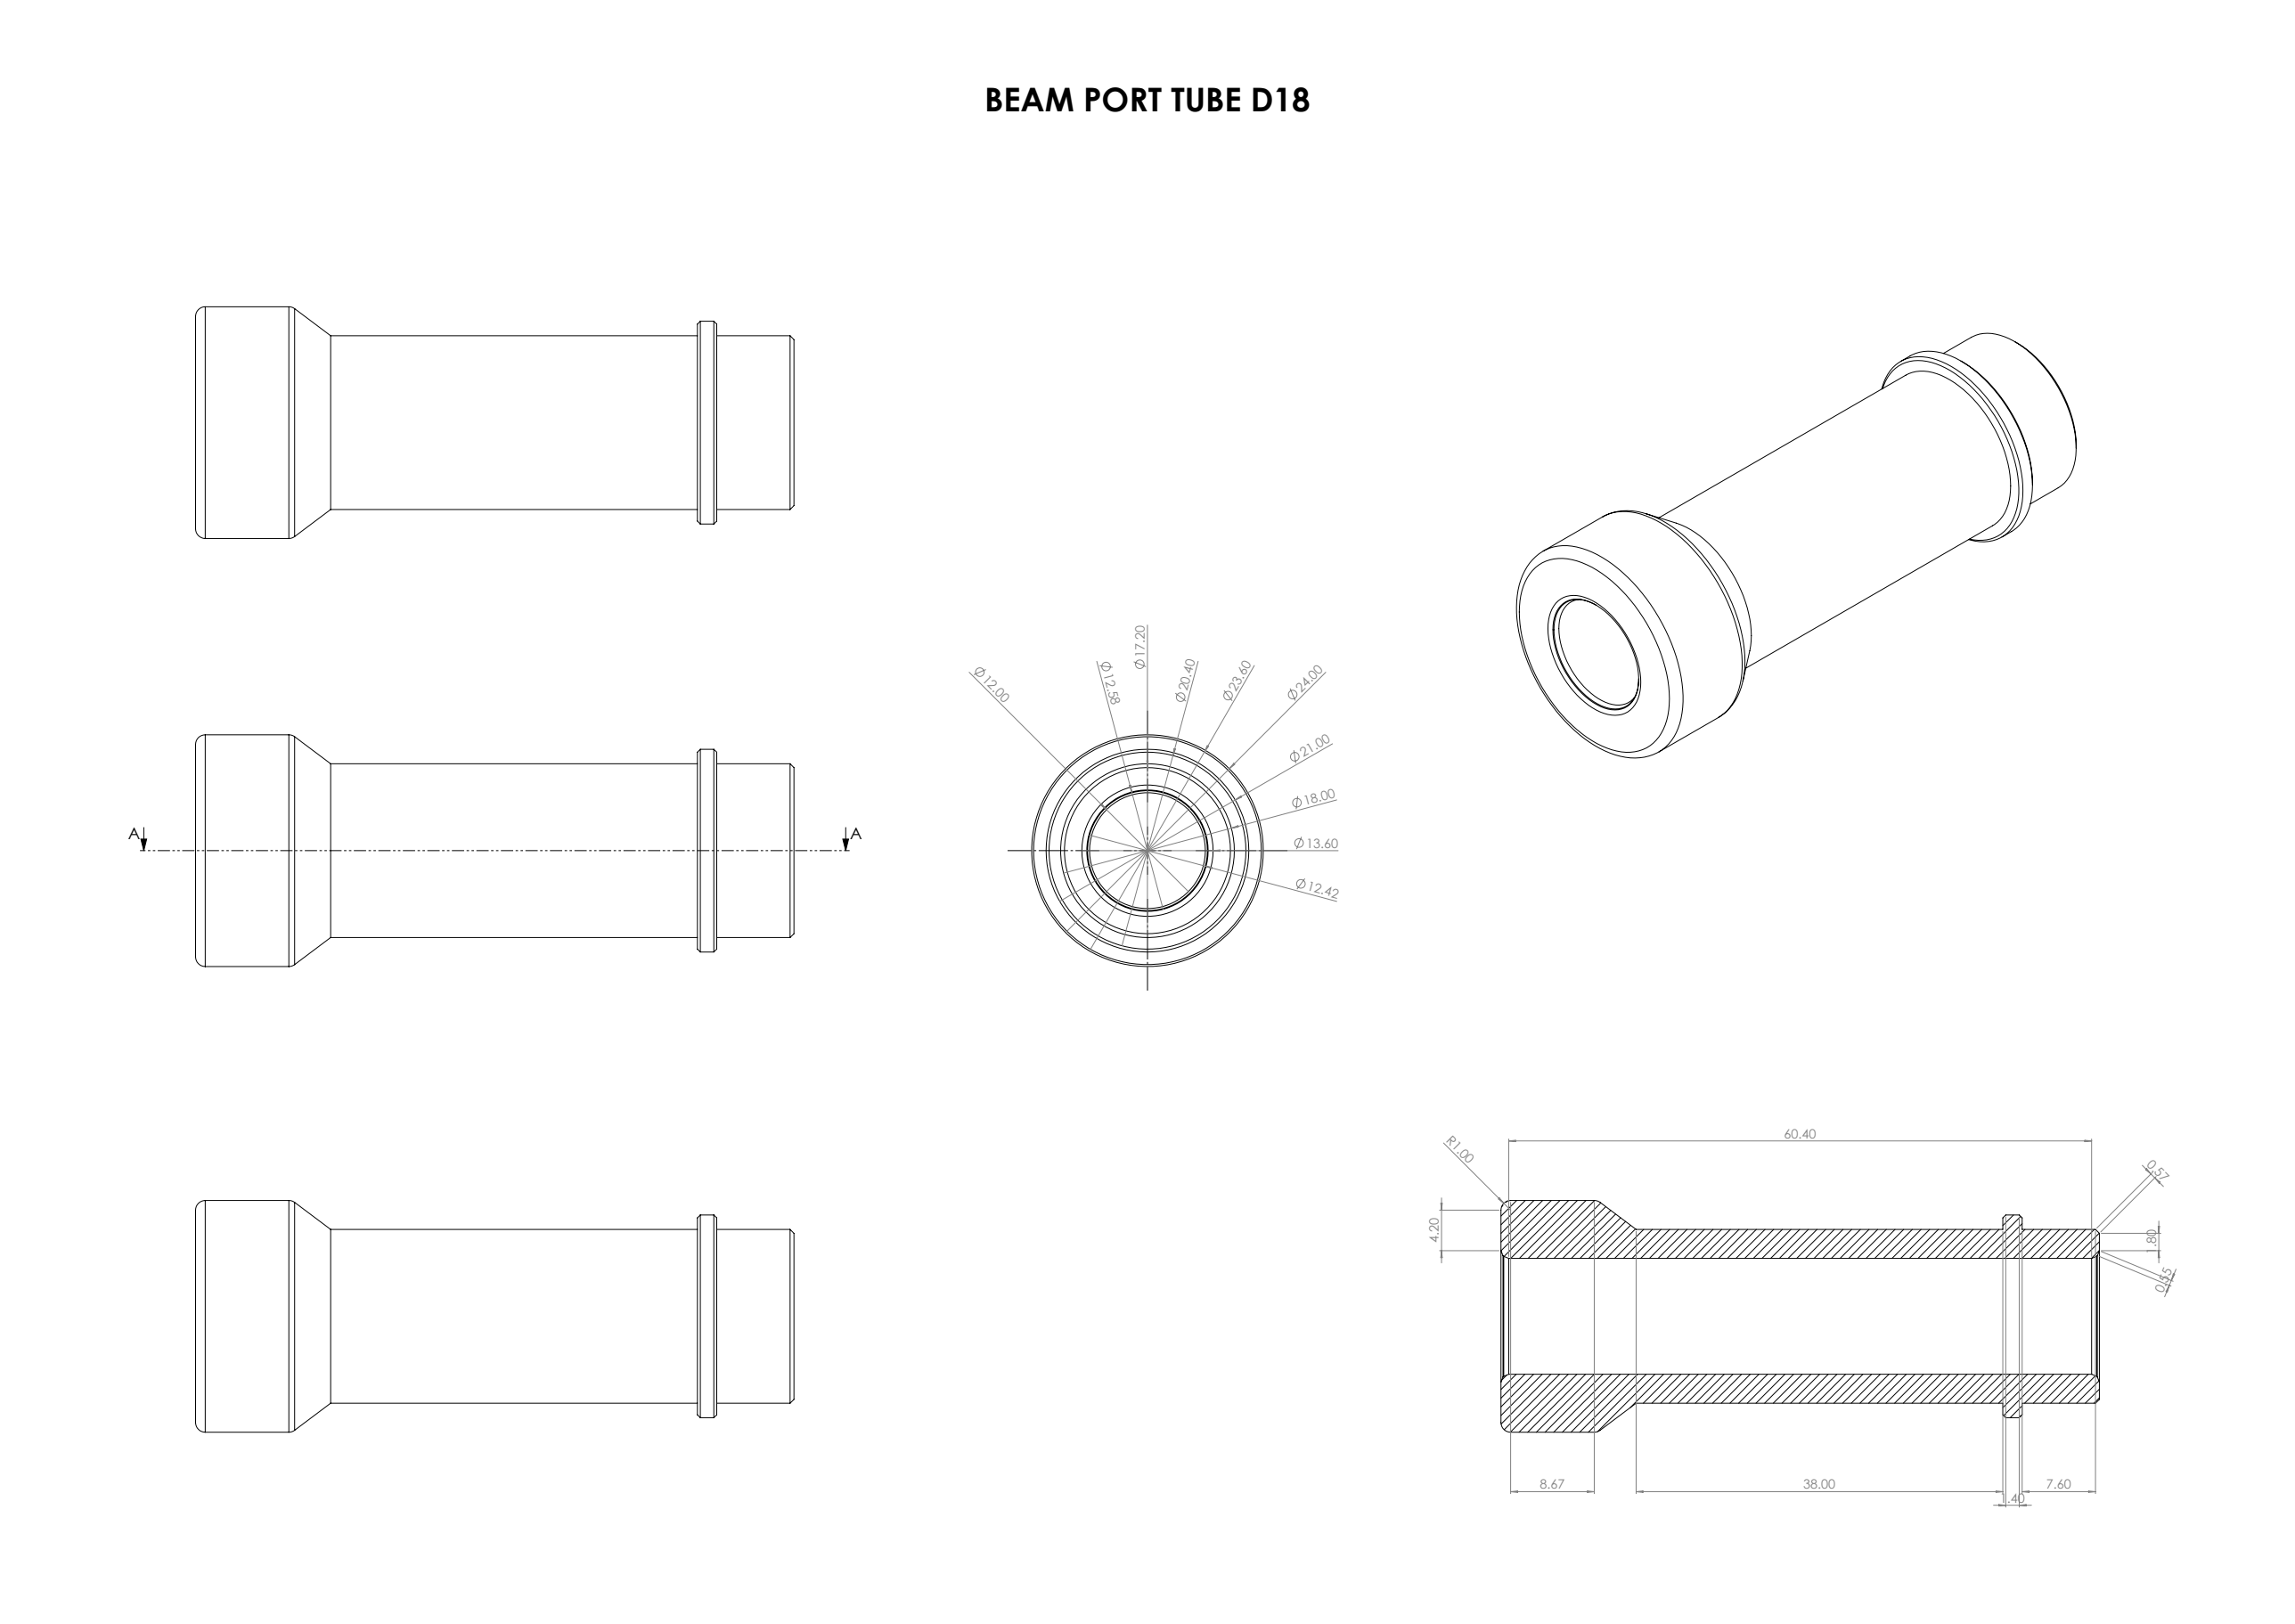
ISO-10303-21;
HEADER;
/* Generated by software containing ST-Developer
 * from STEP Tools, Inc. (www.steptools.com) 
 */

FILE_DESCRIPTION(
/* description */ (''),
/* implementation_level */ '2;1');

FILE_NAME(
/* name */ '04_Beam_Port_Tube_D18.step',
/* time_stamp */ '2026-10-19T23:00:43-07:00',
/* author */ (''),
/* organization */ (''),
/* preprocessor_version */ 'ST-DEVELOPER v20.2',
/* originating_system */ 'Autodesk Translation Framework v15.15.0.0',
/* authorisation */ '');

FILE_SCHEMA (('AUTOMOTIVE_DESIGN { 1 0 10303 214 3 1 1 }'));
ENDSEC;

DATA;
#10=MECHANICAL_DESIGN_GEOMETRIC_PRESENTATION_REPRESENTATION('',(#999),#55002);
#954=TOROIDAL_SURFACE('',#25670,1.1,0.1);
#955=TOROIDAL_SURFACE('',#25675,1.1,0.1);
#959=SHAPE_REPRESENTATION_RELATIONSHIP('SRR','None',#55107,#979);
#979=ADVANCED_BREP_SHAPE_REPRESENTATION('',(#1019),#54985);
#999=STYLED_ITEM('',(#55400),#1019);
#1019=MANIFOLD_SOLID_BREP('Beam Port Tube',#24532);
#1158=FACE_BOUND('',#4320,.T.);
#1159=FACE_BOUND('',#4323,.T.);
#1160=FACE_BOUND('',#4327,.T.);
#1161=FACE_BOUND('',#4334,.T.);
#1414=PLANE('',#25639);
#1415=PLANE('',#25643);
#1416=PLANE('',#25650);
#1417=PLANE('',#25664);
#2116=CYLINDRICAL_SURFACE('',#25636,1.05);
#2117=CYLINDRICAL_SURFACE('',#25655,0.6);
#2118=CYLINDRICAL_SURFACE('',#25669,0.9);
#2119=CYLINDRICAL_SURFACE('',#25673,1.2);
#2120=CYLINDRICAL_SURFACE('',#25680,0.9);
#2831=FACE_OUTER_BOUND('',#4317,.T.);
#2832=FACE_OUTER_BOUND('',#4318,.T.);
#2833=FACE_OUTER_BOUND('',#4319,.T.);
#2834=FACE_OUTER_BOUND('',#4321,.T.);
#2835=FACE_OUTER_BOUND('',#4322,.T.);
#2836=FACE_OUTER_BOUND('',#4324,.T.);
#2837=FACE_OUTER_BOUND('',#4325,.T.);
#2838=FACE_OUTER_BOUND('',#4326,.T.);
#2839=FACE_OUTER_BOUND('',#4328,.T.);
#2840=FACE_OUTER_BOUND('',#4329,.T.);
#2841=FACE_OUTER_BOUND('',#4330,.T.);
#2842=FACE_OUTER_BOUND('',#4331,.T.);
#2843=FACE_OUTER_BOUND('',#4332,.T.);
#2844=FACE_OUTER_BOUND('',#4333,.T.);
#2845=FACE_OUTER_BOUND('',#4335,.T.);
#2846=FACE_OUTER_BOUND('',#4336,.T.);
#2847=FACE_OUTER_BOUND('',#4337,.T.);
#2848=FACE_OUTER_BOUND('',#4338,.T.);
#2849=FACE_OUTER_BOUND('',#4339,.T.);
#2850=FACE_OUTER_BOUND('',#4340,.T.);
#2851=FACE_OUTER_BOUND('',#4341,.T.);
#4317=EDGE_LOOP('',(#17792,#17793,#17794,#17795,#17796));
#4318=EDGE_LOOP('',(#17797,#17798,#17799,#17800,#17801,#17802));
#4319=EDGE_LOOP('',(#17803));
#4320=EDGE_LOOP('',(#17804));
#4321=EDGE_LOOP('',(#17805,#17806,#17807,#17808,#17809));
#4322=EDGE_LOOP('',(#17810));
#4323=EDGE_LOOP('',(#17811));
#4324=EDGE_LOOP('',(#17812,#17813,#17814,#17815));
#4325=EDGE_LOOP('',(#17816,#17817,#17818,#17819));
#4326=EDGE_LOOP('',(#17820));
#4327=EDGE_LOOP('',(#17821));
#4328=EDGE_LOOP('',(#17822,#17823,#17824,#17825,#17826));
#4329=EDGE_LOOP('',(#17827,#17828,#17829,#17830,#17831,#17832));
#4330=EDGE_LOOP('',(#17833,#17834,#17835,#17836,#17837));
#4331=EDGE_LOOP('',(#17838,#17839,#17840,#17841));
#4332=EDGE_LOOP('',(#17842,#17843,#17844,#17845));
#4333=EDGE_LOOP('',(#17846));
#4334=EDGE_LOOP('',(#17847));
#4335=EDGE_LOOP('',(#17848,#17849,#17850,#17851,#17852));
#4336=EDGE_LOOP('',(#17853,#17854,#17855,#17856,#17857));
#4337=EDGE_LOOP('',(#17858,#17859,#17860,#17861));
#4338=EDGE_LOOP('',(#17862,#17863,#17864,#17865));
#4339=EDGE_LOOP('',(#17866,#17867,#17868,#17869));
#4340=EDGE_LOOP('',(#17870,#17871,#17872,#17873));
#4341=EDGE_LOOP('',(#17874,#17875,#17876,#17877));
#5895=LINE('',#35870,#7716);
#5896=LINE('',#35876,#7717);
#5897=LINE('',#35885,#7718);
#5898=LINE('',#35894,#7719);
#5899=LINE('',#35899,#7720);
#5900=LINE('',#35905,#7721);
#5901=LINE('',#35911,#7722);
#5902=LINE('',#35918,#7723);
#5903=LINE('',#35922,#7724);
#5904=LINE('',#35925,#7725);
#5905=LINE('',#35935,#7726);
#5906=LINE('',#35937,#7727);
#5907=LINE('',#35944,#7728);
#5908=LINE('',#35952,#7729);
#5909=LINE('',#35955,#7730);
#7716=VECTOR('',#29439,1.035);
#7717=VECTOR('',#29446,1.05);
#7718=VECTOR('',#29457,1.035);
#7719=VECTOR('',#29468,0.6543933982822);
#7720=VECTOR('',#29475,0.625);
#7721=VECTOR('',#29482,0.610606601717797);
#7722=VECTOR('',#29489,0.6);
#7723=VECTOR('',#29498,0.610606601717798);
#7724=VECTOR('',#29503,0.625);
#7725=VECTOR('',#29506,0.654393398282201);
#7726=VECTOR('',#29519,0.88);
#7727=VECTOR('',#29522,0.9);
#7728=VECTOR('',#29531,1.2);
#7729=VECTOR('',#29542,1.05);
#7730=VECTOR('',#29547,0.9);
#9460=CIRCLE('',#25633,1.02);
#9461=CIRCLE('',#25634,1.05);
#9462=CIRCLE('',#25635,1.05);
#9463=CIRCLE('',#25637,1.05);
#9464=CIRCLE('',#25638,1.05);
#9465=CIRCLE('',#25640,0.9);
#9466=CIRCLE('',#25642,1.02);
#9467=CIRCLE('',#25644,0.9);
#9468=CIRCLE('',#25646,0.628786796564401);
#9469=CIRCLE('',#25647,0.679999999999998);
#9470=CIRCLE('',#25649,0.621213203435595);
#9471=CIRCLE('',#25651,1.1);
#9472=CIRCLE('',#25653,0.6);
#9473=CIRCLE('',#25654,0.6);
#9474=CIRCLE('',#25656,0.6);
#9475=CIRCLE('',#25657,0.6);
#9476=CIRCLE('',#25659,0.621213203435596);
#9477=CIRCLE('',#25661,0.628786796564403);
#9478=CIRCLE('',#25663,0.68);
#9479=CIRCLE('',#25665,0.86);
#9480=CIRCLE('',#25667,0.9);
#9481=CIRCLE('',#25668,0.9);
#9482=CIRCLE('',#25671,0.1);
#9483=CIRCLE('',#25672,1.2);
#9484=CIRCLE('',#25674,1.2);
#9485=CIRCLE('',#25676,0.1);
#9486=CIRCLE('',#25677,1.18);
#9487=CIRCLE('',#25679,0.9);
#10646=VERTEX_POINT('',#35867);
#10647=VERTEX_POINT('',#35869);
#10648=VERTEX_POINT('',#35871);
#10649=VERTEX_POINT('',#35875);
#10650=VERTEX_POINT('',#35877);
#10651=VERTEX_POINT('',#35881);
#10652=VERTEX_POINT('',#35884);
#10653=VERTEX_POINT('',#35888);
#10654=VERTEX_POINT('',#35891);
#10655=VERTEX_POINT('',#35893);
#10656=VERTEX_POINT('',#35897);
#10657=VERTEX_POINT('',#35901);
#10658=VERTEX_POINT('',#35904);
#10659=VERTEX_POINT('',#35906);
#10660=VERTEX_POINT('',#35910);
#10661=VERTEX_POINT('',#35912);
#10662=VERTEX_POINT('',#35916);
#10663=VERTEX_POINT('',#35920);
#10664=VERTEX_POINT('',#35924);
#10665=VERTEX_POINT('',#35928);
#10666=VERTEX_POINT('',#35931);
#10667=VERTEX_POINT('',#35932);
#10668=VERTEX_POINT('',#35939);
#10669=VERTEX_POINT('',#35943);
#10670=VERTEX_POINT('',#35947);
#10671=VERTEX_POINT('',#35951);
#13304=EDGE_CURVE('',#10646,#10646,#9460,.T.);
#13305=EDGE_CURVE('',#10646,#10647,#5895,.T.);
#13306=EDGE_CURVE('',#10647,#10648,#9461,.T.);
#13307=EDGE_CURVE('',#10648,#10647,#9462,.T.);
#13308=EDGE_CURVE('',#10648,#10649,#5896,.T.);
#13309=EDGE_CURVE('',#10650,#10649,#9463,.T.);
#13310=EDGE_CURVE('',#10649,#10650,#9464,.T.);
#13311=EDGE_CURVE('',#10651,#10651,#9465,.T.);
#13312=EDGE_CURVE('',#10650,#10652,#5897,.T.);
#13313=EDGE_CURVE('',#10652,#10652,#9466,.T.);
#13314=EDGE_CURVE('',#10653,#10653,#9467,.T.);
#13315=EDGE_CURVE('',#10654,#10654,#9468,.T.);
#13316=EDGE_CURVE('',#10654,#10655,#5898,.T.);
#13317=EDGE_CURVE('',#10655,#10655,#9469,.T.);
#13318=EDGE_CURVE('',#10656,#10656,#9470,.T.);
#13319=EDGE_CURVE('',#10656,#10654,#5899,.T.);
#13320=EDGE_CURVE('',#10657,#10657,#9471,.T.);
#13321=EDGE_CURVE('',#10656,#10658,#5900,.T.);
#13322=EDGE_CURVE('',#10658,#10659,#9472,.T.);
#13323=EDGE_CURVE('',#10659,#10658,#9473,.T.);
#13324=EDGE_CURVE('',#10659,#10660,#5901,.T.);
#13325=EDGE_CURVE('',#10661,#10660,#9474,.T.);
#13326=EDGE_CURVE('',#10660,#10661,#9475,.T.);
#13327=EDGE_CURVE('',#10662,#10662,#9476,.T.);
#13328=EDGE_CURVE('',#10662,#10661,#5902,.T.);
#13329=EDGE_CURVE('',#10663,#10663,#9477,.T.);
#13330=EDGE_CURVE('',#10663,#10662,#5903,.T.);
#13331=EDGE_CURVE('',#10663,#10664,#5904,.T.);
#13332=EDGE_CURVE('',#10664,#10664,#9478,.T.);
#13333=EDGE_CURVE('',#10665,#10665,#9479,.T.);
#13334=EDGE_CURVE('',#10666,#10667,#9480,.T.);
#13335=EDGE_CURVE('',#10667,#10666,#9481,.T.);
#13336=EDGE_CURVE('',#10666,#10665,#5905,.T.);
#13337=EDGE_CURVE('',#10653,#10667,#5906,.T.);
#13338=EDGE_CURVE('',#10657,#10668,#9482,.T.);
#13339=EDGE_CURVE('',#10668,#10668,#9483,.T.);
#13340=EDGE_CURVE('',#10668,#10669,#5907,.T.);
#13341=EDGE_CURVE('',#10669,#10669,#9484,.T.);
#13342=EDGE_CURVE('',#10669,#10670,#9485,.T.);
#13343=EDGE_CURVE('',#10670,#10670,#9486,.T.);
#13344=EDGE_CURVE('',#10670,#10671,#5908,.T.);
#13345=EDGE_CURVE('',#10671,#10671,#9487,.T.);
#13346=EDGE_CURVE('',#10671,#10651,#5909,.T.);
#17792=ORIENTED_EDGE('',*,*,#13304,.T.);
#17793=ORIENTED_EDGE('',*,*,#13305,.T.);
#17794=ORIENTED_EDGE('',*,*,#13306,.T.);
#17795=ORIENTED_EDGE('',*,*,#13307,.T.);
#17796=ORIENTED_EDGE('',*,*,#13305,.F.);
#17797=ORIENTED_EDGE('',*,*,#13306,.F.);
#17798=ORIENTED_EDGE('',*,*,#13307,.F.);
#17799=ORIENTED_EDGE('',*,*,#13308,.T.);
#17800=ORIENTED_EDGE('',*,*,#13309,.F.);
#17801=ORIENTED_EDGE('',*,*,#13310,.F.);
#17802=ORIENTED_EDGE('',*,*,#13308,.F.);
#17803=ORIENTED_EDGE('',*,*,#13304,.F.);
#17804=ORIENTED_EDGE('',*,*,#13311,.F.);
#17805=ORIENTED_EDGE('',*,*,#13309,.T.);
#17806=ORIENTED_EDGE('',*,*,#13310,.T.);
#17807=ORIENTED_EDGE('',*,*,#13312,.T.);
#17808=ORIENTED_EDGE('',*,*,#13313,.T.);
#17809=ORIENTED_EDGE('',*,*,#13312,.F.);
#17810=ORIENTED_EDGE('',*,*,#13313,.F.);
#17811=ORIENTED_EDGE('',*,*,#13314,.T.);
#17812=ORIENTED_EDGE('',*,*,#13315,.T.);
#17813=ORIENTED_EDGE('',*,*,#13316,.T.);
#17814=ORIENTED_EDGE('',*,*,#13317,.T.);
#17815=ORIENTED_EDGE('',*,*,#13316,.F.);
#17816=ORIENTED_EDGE('',*,*,#13318,.F.);
#17817=ORIENTED_EDGE('',*,*,#13319,.T.);
#17818=ORIENTED_EDGE('',*,*,#13315,.F.);
#17819=ORIENTED_EDGE('',*,*,#13319,.F.);
#17820=ORIENTED_EDGE('',*,*,#13320,.F.);
#17821=ORIENTED_EDGE('',*,*,#13317,.F.);
#17822=ORIENTED_EDGE('',*,*,#13318,.T.);
#17823=ORIENTED_EDGE('',*,*,#13321,.T.);
#17824=ORIENTED_EDGE('',*,*,#13322,.T.);
#17825=ORIENTED_EDGE('',*,*,#13323,.T.);
#17826=ORIENTED_EDGE('',*,*,#13321,.F.);
#17827=ORIENTED_EDGE('',*,*,#13322,.F.);
#17828=ORIENTED_EDGE('',*,*,#13323,.F.);
#17829=ORIENTED_EDGE('',*,*,#13324,.T.);
#17830=ORIENTED_EDGE('',*,*,#13325,.F.);
#17831=ORIENTED_EDGE('',*,*,#13326,.F.);
#17832=ORIENTED_EDGE('',*,*,#13324,.F.);
#17833=ORIENTED_EDGE('',*,*,#13327,.T.);
#17834=ORIENTED_EDGE('',*,*,#13328,.T.);
#17835=ORIENTED_EDGE('',*,*,#13325,.T.);
#17836=ORIENTED_EDGE('',*,*,#13326,.T.);
#17837=ORIENTED_EDGE('',*,*,#13328,.F.);
#17838=ORIENTED_EDGE('',*,*,#13329,.F.);
#17839=ORIENTED_EDGE('',*,*,#13330,.T.);
#17840=ORIENTED_EDGE('',*,*,#13327,.F.);
#17841=ORIENTED_EDGE('',*,*,#13330,.F.);
#17842=ORIENTED_EDGE('',*,*,#13329,.T.);
#17843=ORIENTED_EDGE('',*,*,#13331,.T.);
#17844=ORIENTED_EDGE('',*,*,#13332,.T.);
#17845=ORIENTED_EDGE('',*,*,#13331,.F.);
#17846=ORIENTED_EDGE('',*,*,#13333,.F.);
#17847=ORIENTED_EDGE('',*,*,#13332,.F.);
#17848=ORIENTED_EDGE('',*,*,#13334,.T.);
#17849=ORIENTED_EDGE('',*,*,#13335,.T.);
#17850=ORIENTED_EDGE('',*,*,#13336,.T.);
#17851=ORIENTED_EDGE('',*,*,#13333,.T.);
#17852=ORIENTED_EDGE('',*,*,#13336,.F.);
#17853=ORIENTED_EDGE('',*,*,#13314,.F.);
#17854=ORIENTED_EDGE('',*,*,#13337,.T.);
#17855=ORIENTED_EDGE('',*,*,#13334,.F.);
#17856=ORIENTED_EDGE('',*,*,#13335,.F.);
#17857=ORIENTED_EDGE('',*,*,#13337,.F.);
#17858=ORIENTED_EDGE('',*,*,#13320,.T.);
#17859=ORIENTED_EDGE('',*,*,#13338,.T.);
#17860=ORIENTED_EDGE('',*,*,#13339,.T.);
#17861=ORIENTED_EDGE('',*,*,#13338,.F.);
#17862=ORIENTED_EDGE('',*,*,#13339,.F.);
#17863=ORIENTED_EDGE('',*,*,#13340,.T.);
#17864=ORIENTED_EDGE('',*,*,#13341,.F.);
#17865=ORIENTED_EDGE('',*,*,#13340,.F.);
#17866=ORIENTED_EDGE('',*,*,#13341,.T.);
#17867=ORIENTED_EDGE('',*,*,#13342,.T.);
#17868=ORIENTED_EDGE('',*,*,#13343,.T.);
#17869=ORIENTED_EDGE('',*,*,#13342,.F.);
#17870=ORIENTED_EDGE('',*,*,#13343,.F.);
#17871=ORIENTED_EDGE('',*,*,#13344,.T.);
#17872=ORIENTED_EDGE('',*,*,#13345,.T.);
#17873=ORIENTED_EDGE('',*,*,#13344,.F.);
#17874=ORIENTED_EDGE('',*,*,#13345,.F.);
#17875=ORIENTED_EDGE('',*,*,#13346,.T.);
#17876=ORIENTED_EDGE('',*,*,#13311,.T.);
#17877=ORIENTED_EDGE('',*,*,#13346,.F.);
#23073=CONICAL_SURFACE('',#25632,1.035,0.785398163397459);
#23074=CONICAL_SURFACE('',#25641,1.035,0.785398163397459);
#23075=CONICAL_SURFACE('',#25645,0.6543933982822,1.17809724509617);
#23076=CONICAL_SURFACE('',#25648,0.625,0.785398163397442);
#23077=CONICAL_SURFACE('',#25652,0.610606601717797,0.39269908169869);
#23078=CONICAL_SURFACE('',#25658,0.610606601717798,0.392699081698726);
#23079=CONICAL_SURFACE('',#25660,0.625,0.785398163397442);
#23080=CONICAL_SURFACE('',#25662,0.654393398282201,1.17809724509617);
#23081=CONICAL_SURFACE('',#25666,0.88,0.785398163397459);
#23082=CONICAL_SURFACE('',#25678,1.05,0.643501108793286);
#23584=ADVANCED_FACE('',(#2831),#23073,.T.);
#23585=ADVANCED_FACE('',(#2832),#2116,.T.);
#23586=ADVANCED_FACE('',(#2833,#1158),#1414,.T.);
#23587=ADVANCED_FACE('',(#2834),#23074,.T.);
#23588=ADVANCED_FACE('',(#2835,#1159),#1415,.T.);
#23589=ADVANCED_FACE('',(#2836),#23075,.F.);
#23590=ADVANCED_FACE('',(#2837),#23076,.F.);
#23591=ADVANCED_FACE('',(#2838,#1160),#1416,.T.);
#23592=ADVANCED_FACE('',(#2839),#23077,.F.);
#23593=ADVANCED_FACE('',(#2840),#2117,.F.);
#23594=ADVANCED_FACE('',(#2841),#23078,.F.);
#23595=ADVANCED_FACE('',(#2842),#23079,.F.);
#23596=ADVANCED_FACE('',(#2843),#23080,.F.);
#23597=ADVANCED_FACE('',(#2844,#1161),#1417,.T.);
#23598=ADVANCED_FACE('',(#2845),#23081,.T.);
#23599=ADVANCED_FACE('',(#2846),#2118,.T.);
#23600=ADVANCED_FACE('',(#2847),#954,.T.);
#23601=ADVANCED_FACE('',(#2848),#2119,.T.);
#23602=ADVANCED_FACE('',(#2849),#955,.T.);
#23603=ADVANCED_FACE('',(#2850),#23082,.T.);
#23604=ADVANCED_FACE('',(#2851),#2120,.T.);
#24532=CLOSED_SHELL('',(#23584,#23585,#23586,#23587,#23588,#23589,#23590,
#23591,#23592,#23593,#23594,#23595,#23596,#23597,#23598,#23599,#23600,#23601,
#23602,#23603,#23604));
#25631=AXIS2_PLACEMENT_3D('',#35865,#29433,#29434);
#25632=AXIS2_PLACEMENT_3D('',#35866,#29435,#29436);
#25633=AXIS2_PLACEMENT_3D('',#35868,#29437,#29438);
#25634=AXIS2_PLACEMENT_3D('',#35872,#29440,#29441);
#25635=AXIS2_PLACEMENT_3D('',#35873,#29442,#29443);
#25636=AXIS2_PLACEMENT_3D('',#35874,#29444,#29445);
#25637=AXIS2_PLACEMENT_3D('',#35878,#29447,#29448);
#25638=AXIS2_PLACEMENT_3D('',#35879,#29449,#29450);
#25639=AXIS2_PLACEMENT_3D('',#35880,#29451,#29452);
#25640=AXIS2_PLACEMENT_3D('',#35882,#29453,#29454);
#25641=AXIS2_PLACEMENT_3D('',#35883,#29455,#29456);
#25642=AXIS2_PLACEMENT_3D('',#35886,#29458,#29459);
#25643=AXIS2_PLACEMENT_3D('',#35887,#29460,#29461);
#25644=AXIS2_PLACEMENT_3D('',#35889,#29462,#29463);
#25645=AXIS2_PLACEMENT_3D('',#35890,#29464,#29465);
#25646=AXIS2_PLACEMENT_3D('',#35892,#29466,#29467);
#25647=AXIS2_PLACEMENT_3D('',#35895,#29469,#29470);
#25648=AXIS2_PLACEMENT_3D('',#35896,#29471,#29472);
#25649=AXIS2_PLACEMENT_3D('',#35898,#29473,#29474);
#25650=AXIS2_PLACEMENT_3D('',#35900,#29476,#29477);
#25651=AXIS2_PLACEMENT_3D('',#35902,#29478,#29479);
#25652=AXIS2_PLACEMENT_3D('',#35903,#29480,#29481);
#25653=AXIS2_PLACEMENT_3D('',#35907,#29483,#29484);
#25654=AXIS2_PLACEMENT_3D('',#35908,#29485,#29486);
#25655=AXIS2_PLACEMENT_3D('',#35909,#29487,#29488);
#25656=AXIS2_PLACEMENT_3D('',#35913,#29490,#29491);
#25657=AXIS2_PLACEMENT_3D('',#35914,#29492,#29493);
#25658=AXIS2_PLACEMENT_3D('',#35915,#29494,#29495);
#25659=AXIS2_PLACEMENT_3D('',#35917,#29496,#29497);
#25660=AXIS2_PLACEMENT_3D('',#35919,#29499,#29500);
#25661=AXIS2_PLACEMENT_3D('',#35921,#29501,#29502);
#25662=AXIS2_PLACEMENT_3D('',#35923,#29504,#29505);
#25663=AXIS2_PLACEMENT_3D('',#35926,#29507,#29508);
#25664=AXIS2_PLACEMENT_3D('',#35927,#29509,#29510);
#25665=AXIS2_PLACEMENT_3D('',#35929,#29511,#29512);
#25666=AXIS2_PLACEMENT_3D('',#35930,#29513,#29514);
#25667=AXIS2_PLACEMENT_3D('',#35933,#29515,#29516);
#25668=AXIS2_PLACEMENT_3D('',#35934,#29517,#29518);
#25669=AXIS2_PLACEMENT_3D('',#35936,#29520,#29521);
#25670=AXIS2_PLACEMENT_3D('',#35938,#29523,#29524);
#25671=AXIS2_PLACEMENT_3D('',#35940,#29525,#29526);
#25672=AXIS2_PLACEMENT_3D('',#35941,#29527,#29528);
#25673=AXIS2_PLACEMENT_3D('',#35942,#29529,#29530);
#25674=AXIS2_PLACEMENT_3D('',#35945,#29532,#29533);
#25675=AXIS2_PLACEMENT_3D('',#35946,#29534,#29535);
#25676=AXIS2_PLACEMENT_3D('',#35948,#29536,#29537);
#25677=AXIS2_PLACEMENT_3D('',#35949,#29538,#29539);
#25678=AXIS2_PLACEMENT_3D('',#35950,#29540,#29541);
#25679=AXIS2_PLACEMENT_3D('',#35953,#29543,#29544);
#25680=AXIS2_PLACEMENT_3D('',#35954,#29545,#29546);
#29433=DIRECTION('axis',(0.,0.,1.));
#29434=DIRECTION('refdir',(1.,0.,0.));
#29435=DIRECTION('center_axis',(0.,0.,-1.));
#29436=DIRECTION('ref_axis',(-1.,0.,0.));
#29437=DIRECTION('center_axis',(0.,0.,-1.));
#29438=DIRECTION('ref_axis',(-1.,0.,0.));
#29439=DIRECTION('',(0.707106781186555,8.65956056235503E-17,-0.70710678118654));
#29440=DIRECTION('center_axis',(0.,0.,1.));
#29441=DIRECTION('ref_axis',(-1.,0.,0.));
#29442=DIRECTION('center_axis',(0.,0.,1.));
#29443=DIRECTION('ref_axis',(-1.,0.,0.));
#29444=DIRECTION('center_axis',(0.,0.,1.));
#29445=DIRECTION('ref_axis',(1.,0.,0.));
#29446=DIRECTION('',(0.,0.,-1.));
#29447=DIRECTION('center_axis',(0.,0.,-1.));
#29448=DIRECTION('ref_axis',(-1.,0.,0.));
#29449=DIRECTION('center_axis',(0.,0.,-1.));
#29450=DIRECTION('ref_axis',(-1.,0.,0.));
#29451=DIRECTION('center_axis',(0.,0.,1.));
#29452=DIRECTION('ref_axis',(1.,0.,0.));
#29453=DIRECTION('center_axis',(0.,0.,1.));
#29454=DIRECTION('ref_axis',(1.,0.,0.));
#29455=DIRECTION('center_axis',(0.,0.,1.));
#29456=DIRECTION('ref_axis',(-1.,0.,0.));
#29457=DIRECTION('',(-0.707106781186555,-8.65956056235503E-17,-0.70710678118654));
#29458=DIRECTION('center_axis',(0.,0.,1.));
#29459=DIRECTION('ref_axis',(-1.,0.,0.));
#29460=DIRECTION('center_axis',(0.,0.,-1.));
#29461=DIRECTION('ref_axis',(-1.,0.,0.));
#29462=DIRECTION('center_axis',(0.,0.,1.));
#29463=DIRECTION('ref_axis',(1.,0.,0.));
#29464=DIRECTION('center_axis',(0.,1.81500578188617E-15,1.));
#29465=DIRECTION('ref_axis',(-1.,2.94181504497177E-17,0.));
#29466=DIRECTION('center_axis',(0.,0.,-1.));
#29467=DIRECTION('ref_axis',(-1.,6.12323399573677E-17,0.));
#29468=DIRECTION('',(0.923879532511288,5.54251204061075E-16,0.382683432365087));
#29469=DIRECTION('center_axis',(0.,0.,1.));
#29470=DIRECTION('ref_axis',(-1.,0.,0.));
#29471=DIRECTION('center_axis',(0.,0.,1.));
#29472=DIRECTION('ref_axis',(-1.,0.,0.));
#29473=DIRECTION('center_axis',(0.,0.,1.));
#29474=DIRECTION('ref_axis',(-1.,6.12323399573677E-17,0.));
#29475=DIRECTION('',(0.707106781186543,-8.65956056235487E-17,0.707106781186552));
#29476=DIRECTION('center_axis',(0.,0.,1.));
#29477=DIRECTION('ref_axis',(1.,0.,0.));
#29478=DIRECTION('center_axis',(0.,0.,-1.));
#29479=DIRECTION('ref_axis',(-1.,1.22464679914735E-16,0.));
#29480=DIRECTION('center_axis',(0.,-7.42744751489879E-16,1.));
#29481=DIRECTION('ref_axis',(-1.,3.11479911548302E-17,0.));
#29482=DIRECTION('',(-0.382683432365058,6.51261289894839E-16,-0.9238795325113));
#29483=DIRECTION('center_axis',(0.,0.,-1.));
#29484=DIRECTION('ref_axis',(-1.,0.,0.));
#29485=DIRECTION('center_axis',(0.,0.,-1.));
#29486=DIRECTION('ref_axis',(-1.,0.,0.));
#29487=DIRECTION('center_axis',(0.,0.,1.));
#29488=DIRECTION('ref_axis',(1.,0.,0.));
#29489=DIRECTION('',(0.,0.,-1.));
#29490=DIRECTION('center_axis',(0.,0.,1.));
#29491=DIRECTION('ref_axis',(-1.,0.,0.));
#29492=DIRECTION('center_axis',(0.,0.,1.));
#29493=DIRECTION('ref_axis',(-1.,0.,0.));
#29494=DIRECTION('center_axis',(0.,-7.42744751489906E-16,-1.));
#29495=DIRECTION('ref_axis',(-1.,3.11479911548302E-17,0.));
#29496=DIRECTION('center_axis',(0.,0.,-1.));
#29497=DIRECTION('ref_axis',(-1.,6.12323399573677E-17,0.));
#29498=DIRECTION('',(-0.382683432365092,7.44991698001377E-16,0.923879532511286));
#29499=DIRECTION('center_axis',(0.,0.,-1.));
#29500=DIRECTION('ref_axis',(-1.,0.,0.));
#29501=DIRECTION('center_axis',(0.,0.,1.));
#29502=DIRECTION('ref_axis',(-1.,6.12323399573677E-17,0.));
#29503=DIRECTION('',(-0.707106781186543,8.65956056235487E-17,0.707106781186552));
#29504=DIRECTION('center_axis',(0.,1.81500578188617E-15,-1.));
#29505=DIRECTION('ref_axis',(-1.,2.94181504497177E-17,0.));
#29506=DIRECTION('',(0.923879532511285,7.80536426518631E-16,-0.382683432365095));
#29507=DIRECTION('center_axis',(0.,0.,-1.));
#29508=DIRECTION('ref_axis',(-1.,0.,0.));
#29509=DIRECTION('center_axis',(0.,0.,-1.));
#29510=DIRECTION('ref_axis',(-1.,0.,0.));
#29511=DIRECTION('center_axis',(0.,0.,1.));
#29512=DIRECTION('ref_axis',(-1.,0.,0.));
#29513=DIRECTION('center_axis',(0.,0.,1.));
#29514=DIRECTION('ref_axis',(-1.,0.,0.));
#29515=DIRECTION('center_axis',(0.,0.,-1.));
#29516=DIRECTION('ref_axis',(-1.,0.,0.));
#29517=DIRECTION('center_axis',(0.,0.,-1.));
#29518=DIRECTION('ref_axis',(-1.,0.,0.));
#29519=DIRECTION('',(-0.707106781186555,-8.65956056235503E-17,-0.70710678118654));
#29520=DIRECTION('center_axis',(0.,0.,1.));
#29521=DIRECTION('ref_axis',(1.,0.,0.));
#29522=DIRECTION('',(0.,0.,-1.));
#29523=DIRECTION('center_axis',(0.,0.,1.));
#29524=DIRECTION('ref_axis',(1.,0.,0.));
#29525=DIRECTION('center_axis',(1.22464679914735E-16,-1.,0.));
#29526=DIRECTION('ref_axis',(-1.,-1.22464679914735E-16,0.));
#29527=DIRECTION('center_axis',(0.,0.,1.));
#29528=DIRECTION('ref_axis',(-1.,1.22464679914735E-16,0.));
#29529=DIRECTION('center_axis',(0.,0.,1.));
#29530=DIRECTION('ref_axis',(1.,0.,0.));
#29531=DIRECTION('',(0.,0.,-1.));
#29532=DIRECTION('center_axis',(0.,0.,-1.));
#29533=DIRECTION('ref_axis',(-1.,1.22464679914735E-16,0.));
#29534=DIRECTION('center_axis',(0.,0.,1.));
#29535=DIRECTION('ref_axis',(1.,0.,0.));
#29536=DIRECTION('center_axis',(1.22464679914735E-16,-1.,0.));
#29537=DIRECTION('ref_axis',(-1.,-1.22464679914735E-16,0.));
#29538=DIRECTION('center_axis',(0.,0.,1.));
#29539=DIRECTION('ref_axis',(-1.,0.,0.));
#29540=DIRECTION('center_axis',(0.,0.,1.));
#29541=DIRECTION('ref_axis',(1.,0.,0.));
#29542=DIRECTION('',(0.600000000000001,7.34788079488414E-17,-0.799999999999999));
#29543=DIRECTION('center_axis',(0.,0.,1.));
#29544=DIRECTION('ref_axis',(1.,0.,0.));
#29545=DIRECTION('center_axis',(0.,0.,1.));
#29546=DIRECTION('ref_axis',(1.,0.,0.));
#29547=DIRECTION('',(0.,0.,-1.));
#35865=CARTESIAN_POINT('',(0.,0.,0.));
#35866=CARTESIAN_POINT('Origin',(0.,0.,12.785));
#35867=CARTESIAN_POINT('',(1.02,-1.2491397351303E-16,12.8));
#35868=CARTESIAN_POINT('Origin',(0.,0.,12.8));
#35869=CARTESIAN_POINT('',(1.05,1.28587913910472E-16,12.77));
#35870=CARTESIAN_POINT('',(1.035,1.26750943711751E-16,12.785));
#35871=CARTESIAN_POINT('',(-1.05,-1.28587913910472E-16,12.77));
#35872=CARTESIAN_POINT('Origin',(0.,0.,12.77));
#35873=CARTESIAN_POINT('Origin',(0.,0.,12.77));
#35874=CARTESIAN_POINT('Origin',(0.,0.,12.7));
#35875=CARTESIAN_POINT('',(-1.05,-1.28587913910472E-16,12.63));
#35876=CARTESIAN_POINT('',(-1.05,-1.28587913910472E-16,12.7));
#35877=CARTESIAN_POINT('',(1.05,-1.28587913910472E-16,12.63));
#35878=CARTESIAN_POINT('Origin',(0.,0.,12.63));
#35879=CARTESIAN_POINT('Origin',(0.,0.,12.63));
#35880=CARTESIAN_POINT('Origin',(0.9,0.,12.8));
#35881=CARTESIAN_POINT('',(-0.9,-1.10218211923262E-16,12.8));
#35882=CARTESIAN_POINT('Origin',(0.,0.,12.8));
#35883=CARTESIAN_POINT('Origin',(0.,0.,12.615));
#35884=CARTESIAN_POINT('',(1.02,1.2491397351303E-16,12.6));
#35885=CARTESIAN_POINT('',(1.035,1.26750943711751E-16,12.615));
#35886=CARTESIAN_POINT('Origin',(0.,0.,12.6));
#35887=CARTESIAN_POINT('Origin',(1.05,0.,12.6));
#35888=CARTESIAN_POINT('',(-0.9,-1.10218211923262E-16,12.6));
#35889=CARTESIAN_POINT('Origin',(0.,0.,12.6));
#35890=CARTESIAN_POINT('Origin',(0.,-1.92510434439678E-17,17.9893933982822));
#35891=CARTESIAN_POINT('',(0.628786796564401,-1.54008347551742E-16,17.9787867965644));
#35892=CARTESIAN_POINT('Origin',(0.,-3.85020868879356E-17,17.9787867965644));
#35893=CARTESIAN_POINT('',(0.679999999999998,8.32759823420198E-17,18.));
#35894=CARTESIAN_POINT('',(0.6543933982822,-1.18642164946881E-16,17.9893933982822));
#35895=CARTESIAN_POINT('Origin',(0.,0.,18.));
#35896=CARTESIAN_POINT('Origin',(0.,0.,17.975));
#35897=CARTESIAN_POINT('',(0.621213203435595,0.,17.9712132034356));
#35898=CARTESIAN_POINT('Origin',(0.,-3.80383380587737E-17,17.9712132034356));
#35899=CARTESIAN_POINT('',(0.625,-7.65404249467096E-17,17.975));
#35900=CARTESIAN_POINT('Origin',(0.6,0.,18.));
#35901=CARTESIAN_POINT('',(-1.1,-1.34711147906209E-16,18.));
#35902=CARTESIAN_POINT('Origin',(0.,0.,18.));
#35903=CARTESIAN_POINT('Origin',(0.,-1.90191690293869E-17,17.9456066017178));
#35904=CARTESIAN_POINT('',(0.6,-7.34788079488412E-17,17.92));
#35905=CARTESIAN_POINT('',(0.610606601717797,3.67394039744206E-17,17.9456066017178));
#35906=CARTESIAN_POINT('',(-0.6,-7.34788079488412E-17,17.92));
#35907=CARTESIAN_POINT('Origin',(0.,0.,17.92));
#35908=CARTESIAN_POINT('Origin',(0.,0.,17.92));
#35909=CARTESIAN_POINT('Origin',(0.,0.,14.9));
#35910=CARTESIAN_POINT('',(-0.6,-7.34788079488412E-17,11.88));
#35911=CARTESIAN_POINT('',(-0.6,-7.34788079488412E-17,14.9));
#35912=CARTESIAN_POINT('',(0.6,7.34788079488412E-17,11.88));
#35913=CARTESIAN_POINT('Origin',(0.,0.,11.88));
#35914=CARTESIAN_POINT('Origin',(0.,0.,11.88));
#35915=CARTESIAN_POINT('Origin',(0.,-1.90191690293869E-17,11.8543933982822));
#35916=CARTESIAN_POINT('',(0.621213203435596,-1.52153352235095E-16,11.8287867965644));
#35917=CARTESIAN_POINT('Origin',(0.,-3.80383380587738E-17,11.8287867965644));
#35918=CARTESIAN_POINT('',(0.610606601717798,-1.12816080091968E-16,11.8543933982822));
#35919=CARTESIAN_POINT('Origin',(0.,0.,11.825));
#35920=CARTESIAN_POINT('',(0.628786796564403,0.,11.8212132034356));
#35921=CARTESIAN_POINT('Origin',(0.,-3.85020868879357E-17,11.8212132034356));
#35922=CARTESIAN_POINT('',(0.625,-7.65404249467096E-17,11.825));
#35923=CARTESIAN_POINT('Origin',(0.,-1.92510434439679E-17,11.8106066017178));
#35924=CARTESIAN_POINT('',(0.68,-8.327598234202E-17,11.8));
#35925=CARTESIAN_POINT('',(0.654393398282201,4.163799117101E-17,11.8106066017178));
#35926=CARTESIAN_POINT('Origin',(0.,0.,11.8));
#35927=CARTESIAN_POINT('Origin',(0.9,0.,11.8));
#35928=CARTESIAN_POINT('',(0.86,1.05319624726672E-16,11.8));
#35929=CARTESIAN_POINT('Origin',(0.,0.,11.8));
#35930=CARTESIAN_POINT('Origin',(0.,0.,11.82));
#35931=CARTESIAN_POINT('',(0.9,-1.10218211923262E-16,11.84));
#35932=CARTESIAN_POINT('',(-0.9,-1.10218211923262E-16,11.84));
#35933=CARTESIAN_POINT('Origin',(0.,0.,11.84));
#35934=CARTESIAN_POINT('Origin',(0.,0.,11.84));
#35935=CARTESIAN_POINT('',(0.88,1.07768918324967E-16,11.82));
#35936=CARTESIAN_POINT('Origin',(0.,0.,12.2));
#35937=CARTESIAN_POINT('',(-0.9,-1.10218211923262E-16,12.2));
#35938=CARTESIAN_POINT('Origin',(0.,0.,17.9));
#35939=CARTESIAN_POINT('',(-1.2,-1.46957615897682E-16,17.9));
#35940=CARTESIAN_POINT('Origin',(-1.1,-1.34711147906209E-16,17.9));
#35941=CARTESIAN_POINT('Origin',(0.,0.,17.9));
#35942=CARTESIAN_POINT('Origin',(0.,0.,17.5));
#35943=CARTESIAN_POINT('',(-1.2,-1.46957615897682E-16,17.0333333333333));
#35944=CARTESIAN_POINT('',(-1.2,-1.46957615897682E-16,17.5));
#35945=CARTESIAN_POINT('Origin',(0.,0.,17.0333333333333));
#35946=CARTESIAN_POINT('Origin',(0.,0.,17.0333333333333));
#35947=CARTESIAN_POINT('',(-1.18,-1.44508322299388E-16,16.9733333333333));
#35948=CARTESIAN_POINT('Origin',(-1.1,-1.34711147906209E-16,17.0333333333333));
#35949=CARTESIAN_POINT('Origin',(0.,-1.44508322299388E-16,16.9733333333333));
#35950=CARTESIAN_POINT('Origin',(0.,0.,16.8));
#35951=CARTESIAN_POINT('',(-0.9,-1.10218211923262E-16,16.6));
#35952=CARTESIAN_POINT('',(-1.05,-1.28587913910472E-16,16.8));
#35953=CARTESIAN_POINT('Origin',(0.,0.,16.6));
#35954=CARTESIAN_POINT('Origin',(0.,0.,14.7));
#35955=CARTESIAN_POINT('',(-0.9,-1.10218211923262E-16,14.7));
#54963=UNCERTAINTY_MEASURE_WITH_UNIT(LENGTH_MEASURE(0.001),#55003,
'DISTANCE_ACCURACY_VALUE',
'Maximum model space distance between geometric entities at asserted c
onnectivities');
#54980=UNCERTAINTY_MEASURE_WITH_UNIT(LENGTH_MEASURE(0.001),#55003,
'DISTANCE_ACCURACY_VALUE',
'Maximum model space distance between geometric entities at asserted c
onnectivities');
#54985=(
GEOMETRIC_REPRESENTATION_CONTEXT(3)
GLOBAL_UNCERTAINTY_ASSIGNED_CONTEXT((#54963))
GLOBAL_UNIT_ASSIGNED_CONTEXT((#55003,#55005,#55006))
REPRESENTATION_CONTEXT('','3D')
);
#55002=(
GEOMETRIC_REPRESENTATION_CONTEXT(3)
GLOBAL_UNCERTAINTY_ASSIGNED_CONTEXT((#54980))
GLOBAL_UNIT_ASSIGNED_CONTEXT((#55003,#55005,#55006))
REPRESENTATION_CONTEXT('','3D')
);
#55003=(
LENGTH_UNIT()
NAMED_UNIT(*)
SI_UNIT(.CENTI.,.METRE.)
);
#55005=(
NAMED_UNIT(*)
PLANE_ANGLE_UNIT()
SI_UNIT($,.RADIAN.)
);
#55006=(
NAMED_UNIT(*)
SI_UNIT($,.STERADIAN.)
SOLID_ANGLE_UNIT()
);
#55011=SHAPE_DEFINITION_REPRESENTATION(#55032,#55107);
#55032=PRODUCT_DEFINITION_SHAPE('',$,#55129);
#55107=SHAPE_REPRESENTATION('',(#25631),#54985);
#55124=PRODUCT_DEFINITION_CONTEXT('part definition',#55189,'design');
#55129=PRODUCT_DEFINITION('2026-10-18-23-36-09-603',
'04_Beam_Port_Tube_D18',#55150,#55124);
#55150=PRODUCT_DEFINITION_FORMATION('',$,#55195);
#55189=APPLICATION_CONTEXT(
'Core Data for Automotive Mechanical Design Process');
#55190=PRODUCT_CONTEXT('part definition',#55189,'mechanical');
#55195=PRODUCT('2026-10-18-23-36-09-603','04_Beam_Port_Tube_D18',$,(#55190));
#55394=COLOUR_RGB('Off White',0.89,0.88,0.83);
#55395=FILL_AREA_STYLE_COLOUR('',#55394);
#55396=FILL_AREA_STYLE('',(#55395));
#55397=SURFACE_STYLE_FILL_AREA(#55396);
#55398=SURFACE_SIDE_STYLE('',(#55397));
#55399=SURFACE_STYLE_USAGE(.BOTH.,#55398);
#55400=PRESENTATION_STYLE_ASSIGNMENT((#55399));
ENDSEC;
END-ISO-10303-21;
